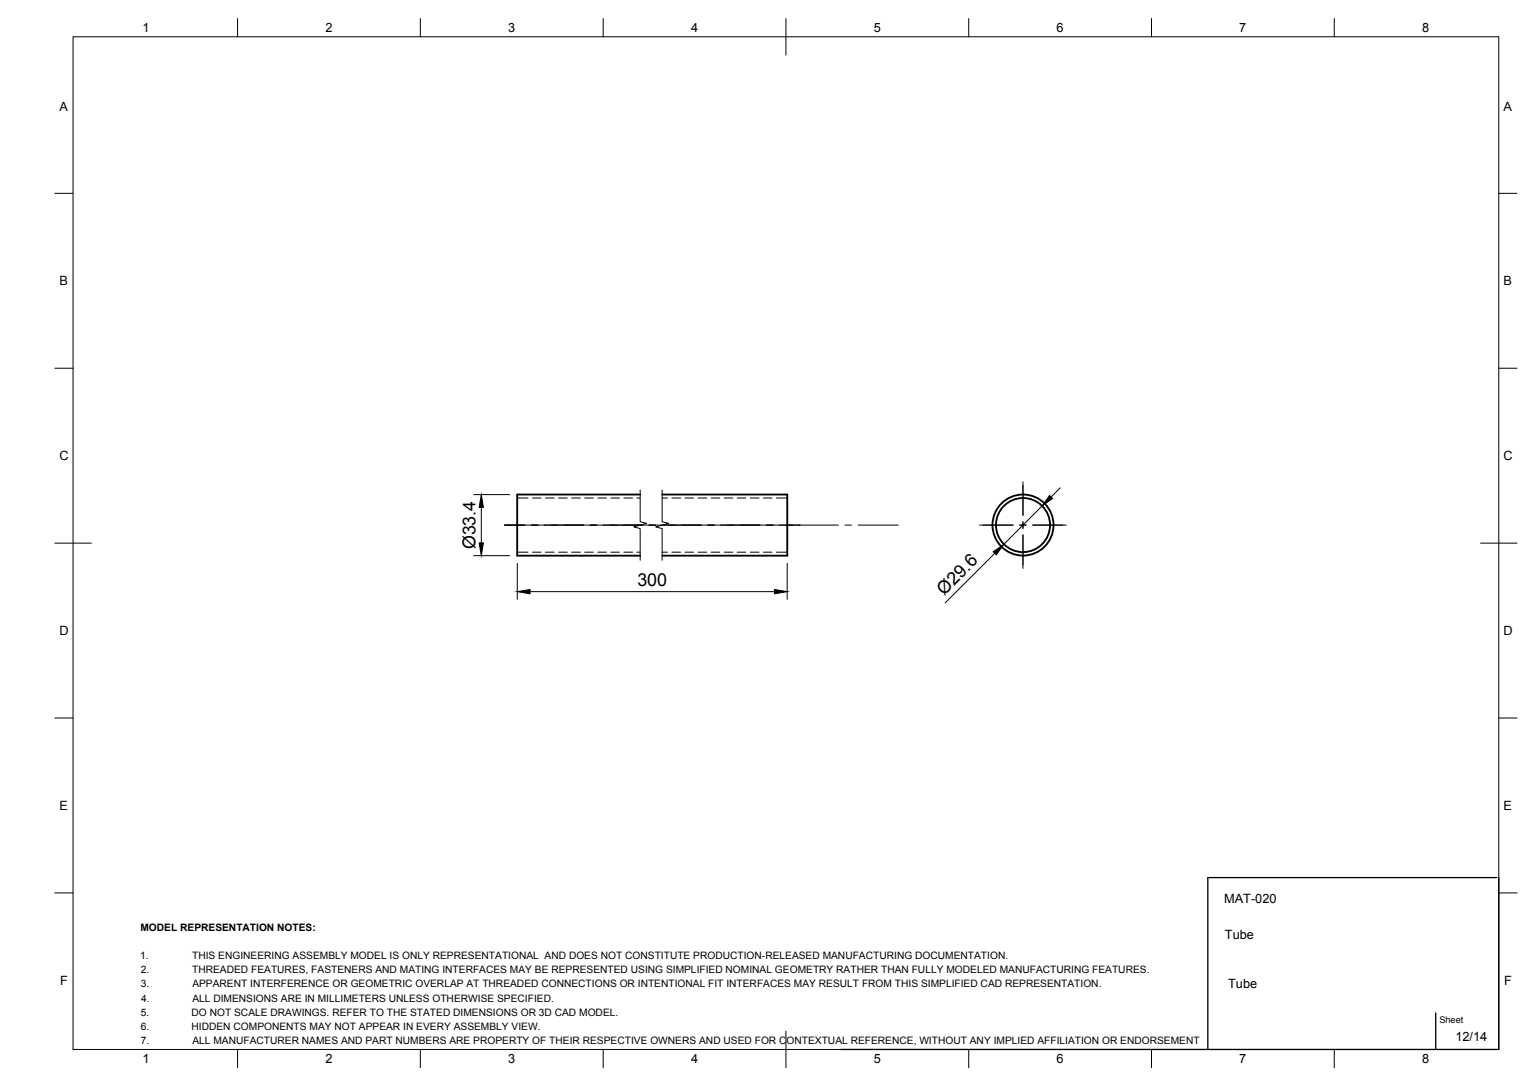
ISO-10303-21;
HEADER;
/* Generated by software containing ST-Developer
 * from STEP Tools, Inc. (www.steptools.com) 
 */

FILE_DESCRIPTION(
/* description */ ('STEP AP214'),
/* implementation_level */ '2;1');

FILE_NAME(
/* name */ 'Tube.step',
/* time_stamp */ '2026-11-14T06:20:50-08:00',
/* author */ (''),
/* organization */ (''),
/* preprocessor_version */ 'ST-DEVELOPER v20.2',
/* originating_system */ 'Autodesk Translation Framework v15.17.0.0',
/* authorisation */ '');

FILE_SCHEMA (('AUTOMOTIVE_DESIGN { 1 0 10303 214 3 1 1 }'));
ENDSEC;

DATA;
#10=MECHANICAL_DESIGN_GEOMETRIC_PRESENTATION_REPRESENTATION('',(#963),#20658);
#134=FACE_BOUND('',#1355,.T.);
#135=FACE_BOUND('',#1357,.T.);
#426=PLANE('',#3988);
#427=PLANE('',#3989);
#595=LINE('',#20328,#788);
#596=LINE('',#20334,#789);
#788=VECTOR('',#4652,14.8);
#789=VECTOR('',#4659,16.7);
#908=CYLINDRICAL_SURFACE('',#3982,14.8);
#909=CYLINDRICAL_SURFACE('',#3985,16.7);
#939=SHAPE_REPRESENTATION_RELATIONSHIP('SRR','None',#20723,#951);
#951=ADVANCED_BREP_SHAPE_REPRESENTATION('',(#975),#20653);
#963=STYLED_ITEM('',(#20787),#975);
#975=MANIFOLD_SOLID_BREP('Body1',#3658);
#1133=FACE_OUTER_BOUND('',#1352,.T.);
#1134=FACE_OUTER_BOUND('',#1353,.T.);
#1135=FACE_OUTER_BOUND('',#1354,.T.);
#1136=FACE_OUTER_BOUND('',#1356,.T.);
#1352=EDGE_LOOP('',(#3218,#3219,#3220,#3221));
#1353=EDGE_LOOP('',(#3222,#3223,#3224,#3225));
#1354=EDGE_LOOP('',(#3226));
#1355=EDGE_LOOP('',(#3227));
#1356=EDGE_LOOP('',(#3228));
#1357=EDGE_LOOP('',(#3229));
#1489=CIRCLE('',#3983,14.8);
#1490=CIRCLE('',#3984,14.8);
#1491=CIRCLE('',#3986,16.7);
#1492=CIRCLE('',#3987,16.7);
#1817=VERTEX_POINT('',#20325);
#1818=VERTEX_POINT('',#20327);
#1819=VERTEX_POINT('',#20331);
#1820=VERTEX_POINT('',#20333);
#2291=EDGE_CURVE('',#1817,#1817,#1489,.T.);
#2292=EDGE_CURVE('',#1817,#1818,#595,.T.);
#2293=EDGE_CURVE('',#1818,#1818,#1490,.T.);
#2294=EDGE_CURVE('',#1819,#1819,#1491,.T.);
#2295=EDGE_CURVE('',#1819,#1820,#596,.T.);
#2296=EDGE_CURVE('',#1820,#1820,#1492,.T.);
#3218=ORIENTED_EDGE('',*,*,#2291,.T.);
#3219=ORIENTED_EDGE('',*,*,#2292,.T.);
#3220=ORIENTED_EDGE('',*,*,#2293,.F.);
#3221=ORIENTED_EDGE('',*,*,#2292,.F.);
#3222=ORIENTED_EDGE('',*,*,#2294,.T.);
#3223=ORIENTED_EDGE('',*,*,#2295,.T.);
#3224=ORIENTED_EDGE('',*,*,#2296,.F.);
#3225=ORIENTED_EDGE('',*,*,#2295,.F.);
#3226=ORIENTED_EDGE('',*,*,#2296,.T.);
#3227=ORIENTED_EDGE('',*,*,#2291,.F.);
#3228=ORIENTED_EDGE('',*,*,#2294,.F.);
#3229=ORIENTED_EDGE('',*,*,#2293,.T.);
#3595=ADVANCED_FACE('',(#1133),#908,.F.);
#3596=ADVANCED_FACE('',(#1134),#909,.T.);
#3597=ADVANCED_FACE('',(#1135,#134),#426,.T.);
#3598=ADVANCED_FACE('',(#1136,#135),#427,.F.);
#3658=CLOSED_SHELL('',(#3595,#3596,#3597,#3598));
#3981=AXIS2_PLACEMENT_3D('',#20323,#4646,#4647);
#3982=AXIS2_PLACEMENT_3D('',#20324,#4648,#4649);
#3983=AXIS2_PLACEMENT_3D('',#20326,#4650,#4651);
#3984=AXIS2_PLACEMENT_3D('',#20329,#4653,#4654);
#3985=AXIS2_PLACEMENT_3D('',#20330,#4655,#4656);
#3986=AXIS2_PLACEMENT_3D('',#20332,#4657,#4658);
#3987=AXIS2_PLACEMENT_3D('',#20335,#4660,#4661);
#3988=AXIS2_PLACEMENT_3D('',#20336,#4662,#4663);
#3989=AXIS2_PLACEMENT_3D('',#20337,#4664,#4665);
#4646=DIRECTION('axis',(0.,0.,1.));
#4647=DIRECTION('refdir',(1.,0.,0.));
#4648=DIRECTION('center_axis',(0.,-1.,0.));
#4649=DIRECTION('ref_axis',(0.,0.,-1.));
#4650=DIRECTION('center_axis',(0.,1.,0.));
#4651=DIRECTION('ref_axis',(0.,0.,1.));
#4652=DIRECTION('',(0.,-1.,0.));
#4653=DIRECTION('center_axis',(0.,1.,0.));
#4654=DIRECTION('ref_axis',(0.,0.,1.));
#4655=DIRECTION('center_axis',(0.,-1.,0.));
#4656=DIRECTION('ref_axis',(0.,0.,-1.));
#4657=DIRECTION('center_axis',(0.,1.,0.));
#4658=DIRECTION('ref_axis',(0.,0.,1.));
#4659=DIRECTION('',(0.,1.,0.));
#4660=DIRECTION('center_axis',(0.,1.,0.));
#4661=DIRECTION('ref_axis',(0.,0.,1.));
#4662=DIRECTION('center_axis',(0.,1.,0.));
#4663=DIRECTION('ref_axis',(0.,0.,1.));
#4664=DIRECTION('center_axis',(0.,1.,0.));
#4665=DIRECTION('ref_axis',(0.,0.,1.));
#20323=CARTESIAN_POINT('',(0.,0.,0.));
#20324=CARTESIAN_POINT('Origin',(0.,300.,0.));
#20325=CARTESIAN_POINT('',(-1.81247726273808E-15,300.,14.8));
#20326=CARTESIAN_POINT('Origin',(0.,300.,0.));
#20327=CARTESIAN_POINT('',(-1.81247726273808E-15,0.,14.8));
#20328=CARTESIAN_POINT('',(-1.81247726273808E-15,300.,14.8));
#20329=CARTESIAN_POINT('Origin',(0.,0.,0.));
#20330=CARTESIAN_POINT('Origin',(0.,300.,0.));
#20331=CARTESIAN_POINT('',(-2.04516015457608E-15,0.,16.7));
#20332=CARTESIAN_POINT('Origin',(0.,0.,0.));
#20333=CARTESIAN_POINT('',(-2.04516015457608E-15,300.,16.7));
#20334=CARTESIAN_POINT('',(-2.04516015457608E-15,300.,16.7));
#20335=CARTESIAN_POINT('Origin',(0.,300.,0.));
#20336=CARTESIAN_POINT('Origin',(0.,300.,0.));
#20337=CARTESIAN_POINT('Origin',(0.,0.,0.));
#20639=UNCERTAINTY_MEASURE_WITH_UNIT(LENGTH_MEASURE(0.01),#20659,
'DISTANCE_ACCURACY_VALUE',
'Maximum model space distance between geometric entities at asserted c
onnectivities');
#20644=UNCERTAINTY_MEASURE_WITH_UNIT(LENGTH_MEASURE(0.01),#20659,
'DISTANCE_ACCURACY_VALUE',
'Maximum model space distance between geometric entities at asserted c
onnectivities');
#20653=(
GEOMETRIC_REPRESENTATION_CONTEXT(3)
GLOBAL_UNCERTAINTY_ASSIGNED_CONTEXT((#20639))
GLOBAL_UNIT_ASSIGNED_CONTEXT((#20659,#20661,#20662))
REPRESENTATION_CONTEXT('','3D')
);
#20658=(
GEOMETRIC_REPRESENTATION_CONTEXT(3)
GLOBAL_UNCERTAINTY_ASSIGNED_CONTEXT((#20644))
GLOBAL_UNIT_ASSIGNED_CONTEXT((#20659,#20661,#20662))
REPRESENTATION_CONTEXT('','3D')
);
#20659=(
LENGTH_UNIT()
NAMED_UNIT(*)
SI_UNIT(.MILLI.,.METRE.)
);
#20661=(
NAMED_UNIT(*)
PLANE_ANGLE_UNIT()
SI_UNIT($,.RADIAN.)
);
#20662=(
NAMED_UNIT(*)
SI_UNIT($,.STERADIAN.)
SOLID_ANGLE_UNIT()
);
#20671=SHAPE_DEFINITION_REPRESENTATION(#20684,#20723);
#20684=PRODUCT_DEFINITION_SHAPE('',$,#20737);
#20723=SHAPE_REPRESENTATION('',(#3981),#20653);
#20728=PRODUCT_DEFINITION_CONTEXT('part definition',#20769,'design');
#20737=PRODUCT_DEFINITION('Tube','Tube',#20750,#20728);
#20750=PRODUCT_DEFINITION_FORMATION('',$,#20779);
#20769=APPLICATION_CONTEXT(
'Core Data for Automotive Mechanical Design Process');
#20770=PRODUCT_CONTEXT('part definition',#20769,'mechanical');
#20779=PRODUCT('Tube','Tube',$,(#20770));
#20787=PRESENTATION_STYLE_ASSIGNMENT((#20792));
#20792=SURFACE_STYLE_USAGE(.BOTH.,#20797);
#20797=SURFACE_SIDE_STYLE('',(#20802));
#20802=SURFACE_STYLE_FILL_AREA(#20807);
#20807=FILL_AREA_STYLE('Opaque(227,224,212)',(#20812));
#20812=FILL_AREA_STYLE_COLOUR('Opaque(227,224,212)',#20817);
#20817=COLOUR_RGB('Opaque(227,224,212)',0.890196078431372,0.87843137254902,
0.831372549019608);
ENDSEC;
END-ISO-10303-21;
